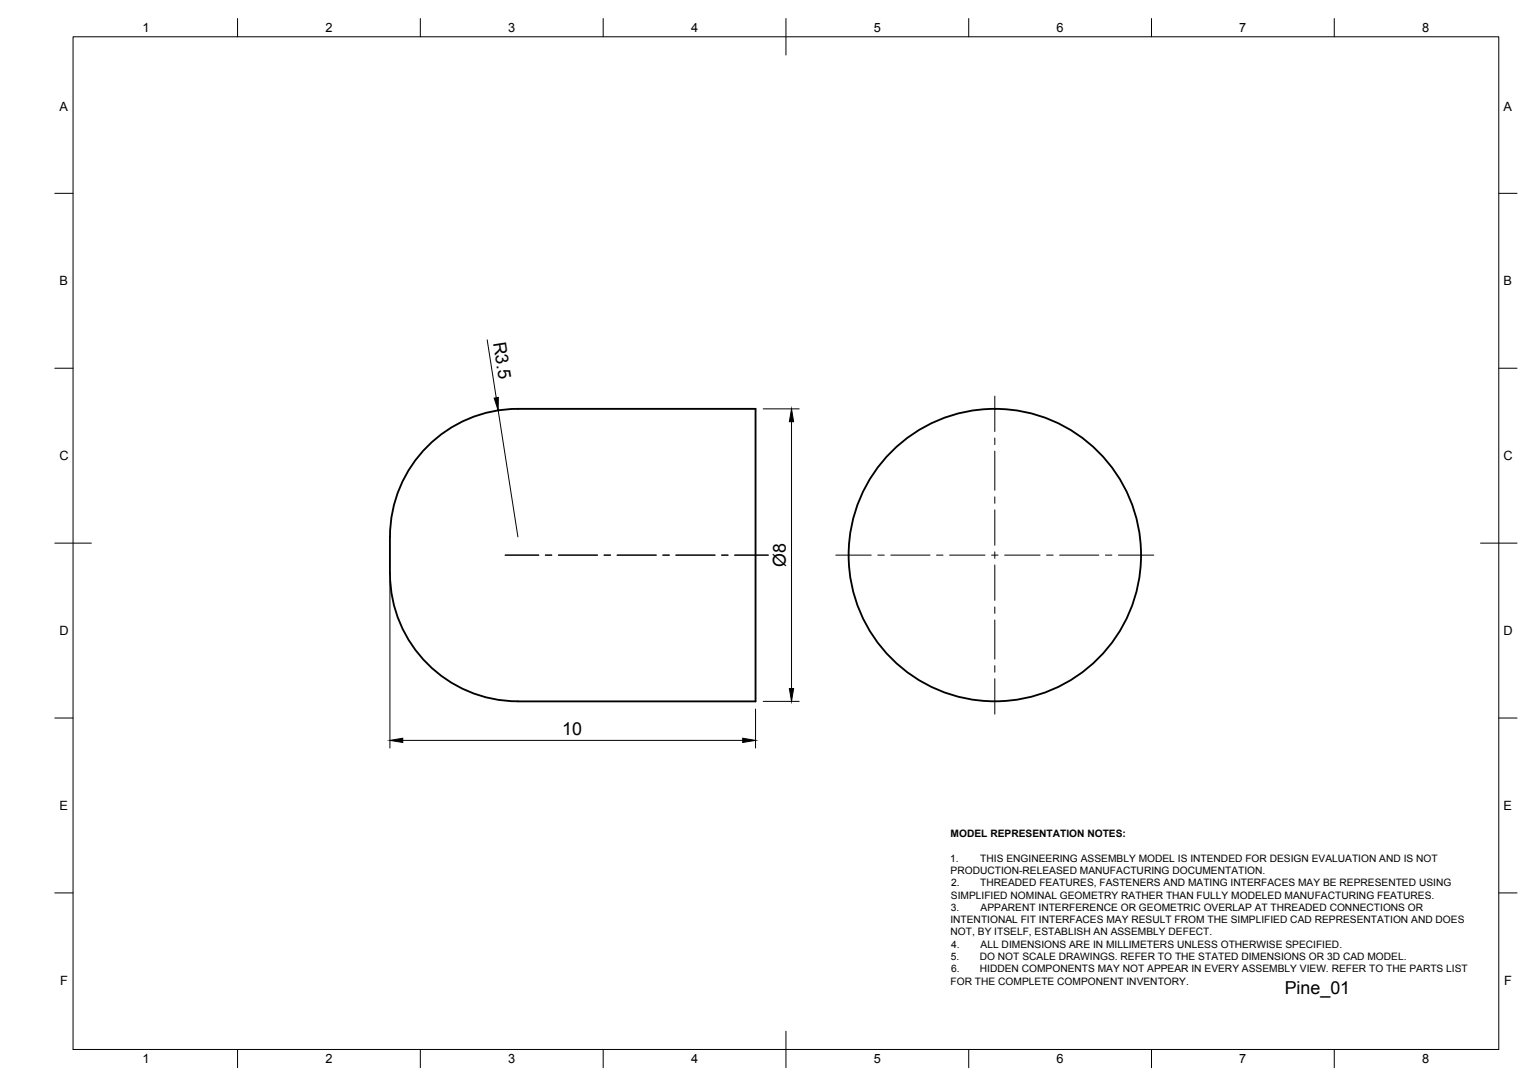
ISO-10303-21;
HEADER;
/* Generated by software containing ST-Developer
 * from STEP Tools, Inc. (www.steptools.com) 
 */

FILE_DESCRIPTION(
/* description */ (''),
/* implementation_level */ '2;1');

FILE_NAME(
/* name */ 'Pine_01.step',
/* time_stamp */ '2026-10-06T13:31:15-07:00',
/* author */ (''),
/* organization */ (''),
/* preprocessor_version */ 'ST-DEVELOPER v20.2',
/* originating_system */ 'Autodesk Translation Framework v15.15.0.0',
/* authorisation */ '');

FILE_SCHEMA (('AUTOMOTIVE_DESIGN { 1 0 10303 214 3 1 1 }'));
ENDSEC;

DATA;
#10=MECHANICAL_DESIGN_GEOMETRIC_PRESENTATION_REPRESENTATION('',(#86),#3154);
#50=(
BOUNDED_SURFACE()
B_SPLINE_SURFACE(2,2,((#2568,#2569,#2570,#2571,#2572,#2573,#2574,#2575,
#2576),(#2577,#2578,#2579,#2580,#2581,#2582,#2583,#2584,#2585),(#2586,#2587,
#2588,#2589,#2590,#2591,#2592,#2593,#2594)),.UNSPECIFIED.,.F.,.T.,.F.)
B_SPLINE_SURFACE_WITH_KNOTS((3,3),(3,2,2,2,3),(-1.96675441490332E-13,1.57079632679509),
(-3.14159265358979,-1.5707963267949,0.,1.5707963267949,3.14159265358979),
 .UNSPECIFIED.)
GEOMETRIC_REPRESENTATION_ITEM()
RATIONAL_B_SPLINE_SURFACE(((1.,0.707106781186548,1.,0.707106781186548,1.,
0.707106781186548,1.,0.707106781186548,1.),(0.707106781186405,0.499999999999899,
0.707106781186405,0.499999999999899,0.707106781186405,0.499999999999899,
0.707106781186405,0.499999999999899,0.707106781186405),(1.,0.707106781186548,
1.,0.707106781186548,1.,0.707106781186548,1.,0.707106781186548,1.)))
REPRESENTATION_ITEM('')
SURFACE()
);
#68=SHAPE_REPRESENTATION_RELATIONSHIP('SRR','None',#3196,#77);
#77=ADVANCED_BREP_SHAPE_REPRESENTATION('',(#95),#3152);
#86=STYLED_ITEM('',(#3243),#95);
#95=MANIFOLD_SOLID_BREP('Body1',#1088);
#124=PLANE('',#1264);
#125=PLANE('',#1265);
#162=CIRCLE('',#1258,3.99999999999999);
#163=CIRCLE('',#1259,3.49999999999994);
#164=CIRCLE('',#1260,0.49999999999999);
#165=CIRCLE('',#1261,3.99999999999999);
#166=CIRCLE('',#1263,3.99999999999999);
#218=FACE_OUTER_BOUND('',#282,.T.);
#219=FACE_OUTER_BOUND('',#283,.T.);
#220=FACE_OUTER_BOUND('',#284,.T.);
#221=FACE_OUTER_BOUND('',#285,.T.);
#282=EDGE_LOOP('',(#928,#929,#930,#931,#932));
#283=EDGE_LOOP('',(#933,#934,#935,#936,#937));
#284=EDGE_LOOP('',(#938));
#285=EDGE_LOOP('',(#939));
#355=LINE('',#2604,#421);
#421=VECTOR('',#1487,3.99999999999999);
#548=VERTEX_POINT('',#2595);
#549=VERTEX_POINT('',#2596);
#550=VERTEX_POINT('',#2598);
#551=VERTEX_POINT('',#2603);
#680=EDGE_CURVE('',#548,#549,#162,.T.);
#681=EDGE_CURVE('',#549,#550,#163,.T.);
#682=EDGE_CURVE('',#550,#550,#164,.T.);
#683=EDGE_CURVE('',#549,#548,#165,.T.);
#684=EDGE_CURVE('',#548,#551,#355,.T.);
#685=EDGE_CURVE('',#551,#551,#166,.T.);
#928=ORIENTED_EDGE('',*,*,#680,.T.);
#929=ORIENTED_EDGE('',*,*,#681,.T.);
#930=ORIENTED_EDGE('',*,*,#682,.T.);
#931=ORIENTED_EDGE('',*,*,#681,.F.);
#932=ORIENTED_EDGE('',*,*,#683,.T.);
#933=ORIENTED_EDGE('',*,*,#680,.F.);
#934=ORIENTED_EDGE('',*,*,#684,.T.);
#935=ORIENTED_EDGE('',*,*,#685,.T.);
#936=ORIENTED_EDGE('',*,*,#684,.F.);
#937=ORIENTED_EDGE('',*,*,#683,.F.);
#938=ORIENTED_EDGE('',*,*,#682,.F.);
#939=ORIENTED_EDGE('',*,*,#685,.F.);
#1017=CYLINDRICAL_SURFACE('',#1262,3.99999999999999);
#1069=ADVANCED_FACE('',(#218),#50,.F.);
#1070=ADVANCED_FACE('',(#219),#1017,.T.);
#1071=ADVANCED_FACE('',(#220),#124,.T.);
#1072=ADVANCED_FACE('',(#221),#125,.F.);
#1088=CLOSED_SHELL('',(#1069,#1070,#1071,#1072));
#1257=AXIS2_PLACEMENT_3D('',#2567,#1475,#1476);
#1258=AXIS2_PLACEMENT_3D('',#2597,#1477,#1478);
#1259=AXIS2_PLACEMENT_3D('',#2599,#1479,#1480);
#1260=AXIS2_PLACEMENT_3D('',#2600,#1481,#1482);
#1261=AXIS2_PLACEMENT_3D('',#2601,#1483,#1484);
#1262=AXIS2_PLACEMENT_3D('',#2602,#1485,#1486);
#1263=AXIS2_PLACEMENT_3D('',#2605,#1488,#1489);
#1264=AXIS2_PLACEMENT_3D('',#2606,#1490,#1491);
#1265=AXIS2_PLACEMENT_3D('',#2607,#1492,#1493);
#1475=DIRECTION('axis',(0.,0.,1.));
#1476=DIRECTION('refdir',(1.,0.,0.));
#1477=DIRECTION('center_axis',(1.,0.,0.));
#1478=DIRECTION('ref_axis',(0.,1.,0.));
#1479=DIRECTION('center_axis',(-3.42164774028179E-14,1.,1.22464679909721E-16));
#1480=DIRECTION('ref_axis',(-1.46549439250521E-13,-1.22464679914735E-16,
1.));
#1481=DIRECTION('center_axis',(-1.,0.,0.));
#1482=DIRECTION('ref_axis',(0.,1.,0.));
#1483=DIRECTION('center_axis',(1.,0.,0.));
#1484=DIRECTION('ref_axis',(0.,1.,0.));
#1485=DIRECTION('center_axis',(1.,0.,0.));
#1486=DIRECTION('ref_axis',(0.,1.,0.));
#1487=DIRECTION('',(-1.,0.,0.));
#1488=DIRECTION('center_axis',(1.,0.,0.));
#1489=DIRECTION('ref_axis',(0.,1.,0.));
#1490=DIRECTION('center_axis',(1.,0.,0.));
#1491=DIRECTION('ref_axis',(0.,1.,0.));
#1492=DIRECTION('center_axis',(1.,0.,0.));
#1493=DIRECTION('ref_axis',(0.,1.,0.));
#2567=CARTESIAN_POINT('',(0.,0.,0.));
#2568=CARTESIAN_POINT('Ctrl Pts',(21.4999999999988,1.86764666232119E-14,
184.));
#2569=CARTESIAN_POINT('Ctrl Pts',(21.4999999999989,-3.99999999999997,184.));
#2570=CARTESIAN_POINT('Ctrl Pts',(21.4999999999995,-3.99999999999997,180.));
#2571=CARTESIAN_POINT('Ctrl Pts',(21.5000000000001,-3.99999999999997,176.));
#2572=CARTESIAN_POINT('Ctrl Pts',(21.5,1.86764666232117E-14,176.));
#2573=CARTESIAN_POINT('Ctrl Pts',(21.4999999999998,4.,176.));
#2574=CARTESIAN_POINT('Ctrl Pts',(21.4999999999992,4.,180.));
#2575=CARTESIAN_POINT('Ctrl Pts',(21.4999999999986,4.,184.));
#2576=CARTESIAN_POINT('Ctrl Pts',(21.4999999999988,1.86764666232119E-14,
184.));
#2577=CARTESIAN_POINT('Ctrl Pts',(25.0000000000001,1.38434137533119E-13,
184.000000000001));
#2578=CARTESIAN_POINT('Ctrl Pts',(25.0000000000002,-4.00000000000052,184.000000000001));
#2579=CARTESIAN_POINT('Ctrl Pts',(25.0000000000008,-4.00000000000052,180.000000000001));
#2580=CARTESIAN_POINT('Ctrl Pts',(25.0000000000014,-4.00000000000052,176.));
#2581=CARTESIAN_POINT('Ctrl Pts',(25.0000000000013,1.38434137533119E-13,
176.));
#2582=CARTESIAN_POINT('Ctrl Pts',(25.0000000000011,4.0000000000008,176.));
#2583=CARTESIAN_POINT('Ctrl Pts',(25.0000000000005,4.0000000000008,180.000000000001));
#2584=CARTESIAN_POINT('Ctrl Pts',(25.,4.0000000000008,184.000000000001));
#2585=CARTESIAN_POINT('Ctrl Pts',(25.0000000000001,1.38434137533119E-13,
184.000000000001));
#2586=CARTESIAN_POINT('Ctrl Pts',(24.9999999999999,1.38434137533096E-13,
180.5));
#2587=CARTESIAN_POINT('Ctrl Pts',(24.9999999999999,-0.499999999999194,180.5));
#2588=CARTESIAN_POINT('Ctrl Pts',(25.,-0.499999999999194,180.000000000001));
#2589=CARTESIAN_POINT('Ctrl Pts',(25.0000000000001,-0.499999999999194,179.500000000001));
#2590=CARTESIAN_POINT('Ctrl Pts',(25.0000000000001,1.38434137533096E-13,
179.500000000001));
#2591=CARTESIAN_POINT('Ctrl Pts',(25.0000000000001,0.49999999999947,179.500000000001));
#2592=CARTESIAN_POINT('Ctrl Pts',(25.,0.499999999999471,180.000000000001));
#2593=CARTESIAN_POINT('Ctrl Pts',(24.9999999999999,0.49999999999947,180.5));
#2594=CARTESIAN_POINT('Ctrl Pts',(24.9999999999999,1.38434137533096E-13,
180.5));
#2595=CARTESIAN_POINT('',(21.5,-3.99999999999999,180.));
#2596=CARTESIAN_POINT('',(21.5,1.81866079035945E-14,184.));
#2597=CARTESIAN_POINT('Origin',(21.5,0.,180.));
#2598=CARTESIAN_POINT('',(25.,-6.12323399573644E-17,180.5));
#2599=CARTESIAN_POINT('Origin',(21.5,1.86152342832779E-14,180.5));
#2600=CARTESIAN_POINT('Origin',(25.,0.,180.));
#2601=CARTESIAN_POINT('Origin',(21.5,0.,180.));
#2602=CARTESIAN_POINT('Origin',(0.,0.,180.));
#2603=CARTESIAN_POINT('',(15.,-3.99999999999999,180.));
#2604=CARTESIAN_POINT('',(0.,-3.99999999999999,180.));
#2605=CARTESIAN_POINT('Origin',(15.,0.,180.));
#2606=CARTESIAN_POINT('Origin',(25.,0.,180.));
#2607=CARTESIAN_POINT('Origin',(15.,0.,180.));
#3141=UNCERTAINTY_MEASURE_WITH_UNIT(LENGTH_MEASURE(0.01),#3155,
'DISTANCE_ACCURACY_VALUE',
'Maximum model space distance between geometric entities at asserted c
onnectivities');
#3143=UNCERTAINTY_MEASURE_WITH_UNIT(LENGTH_MEASURE(0.01),#3155,
'DISTANCE_ACCURACY_VALUE',
'Maximum model space distance between geometric entities at asserted c
onnectivities');
#3152=(
GEOMETRIC_REPRESENTATION_CONTEXT(3)
GLOBAL_UNCERTAINTY_ASSIGNED_CONTEXT((#3141))
GLOBAL_UNIT_ASSIGNED_CONTEXT((#3155,#3157,#3158))
REPRESENTATION_CONTEXT('','3D')
);
#3154=(
GEOMETRIC_REPRESENTATION_CONTEXT(3)
GLOBAL_UNCERTAINTY_ASSIGNED_CONTEXT((#3143))
GLOBAL_UNIT_ASSIGNED_CONTEXT((#3155,#3157,#3158))
REPRESENTATION_CONTEXT('','3D')
);
#3155=(
LENGTH_UNIT()
NAMED_UNIT(*)
SI_UNIT(.MILLI.,.METRE.)
);
#3157=(
NAMED_UNIT(*)
PLANE_ANGLE_UNIT()
SI_UNIT($,.RADIAN.)
);
#3158=(
NAMED_UNIT(*)
SI_UNIT($,.STERADIAN.)
SOLID_ANGLE_UNIT()
);
#3167=SHAPE_DEFINITION_REPRESENTATION(#3177,#3196);
#3177=PRODUCT_DEFINITION_SHAPE('',$,#3207);
#3196=SHAPE_REPRESENTATION('',(#1257),#3152);
#3198=PRODUCT_DEFINITION_CONTEXT('part definition',#3230,'design');
#3207=PRODUCT_DEFINITION('Pine_01','Pine_01',#3217,#3198);
#3217=PRODUCT_DEFINITION_FORMATION('',$,#3240);
#3230=APPLICATION_CONTEXT(
'Core Data for Automotive Mechanical Design Process');
#3231=PRODUCT_CONTEXT('part definition',#3230,'mechanical');
#3240=PRODUCT('Pine_01','Pine_01',$,(#3231));
#3243=PRESENTATION_STYLE_ASSIGNMENT((#3245));
#3245=SURFACE_STYLE_USAGE(.BOTH.,#3247);
#3247=SURFACE_SIDE_STYLE('',(#3249));
#3249=SURFACE_STYLE_FILL_AREA(#3251);
#3251=FILL_AREA_STYLE('Opaque(160,160,160)',(#3253));
#3253=FILL_AREA_STYLE_COLOUR('Opaque(160,160,160)',#3255);
#3255=COLOUR_RGB('Opaque(160,160,160)', 0.09019608, 0.27058824, 0.51372549);
ENDSEC;
END-ISO-10303-21;
